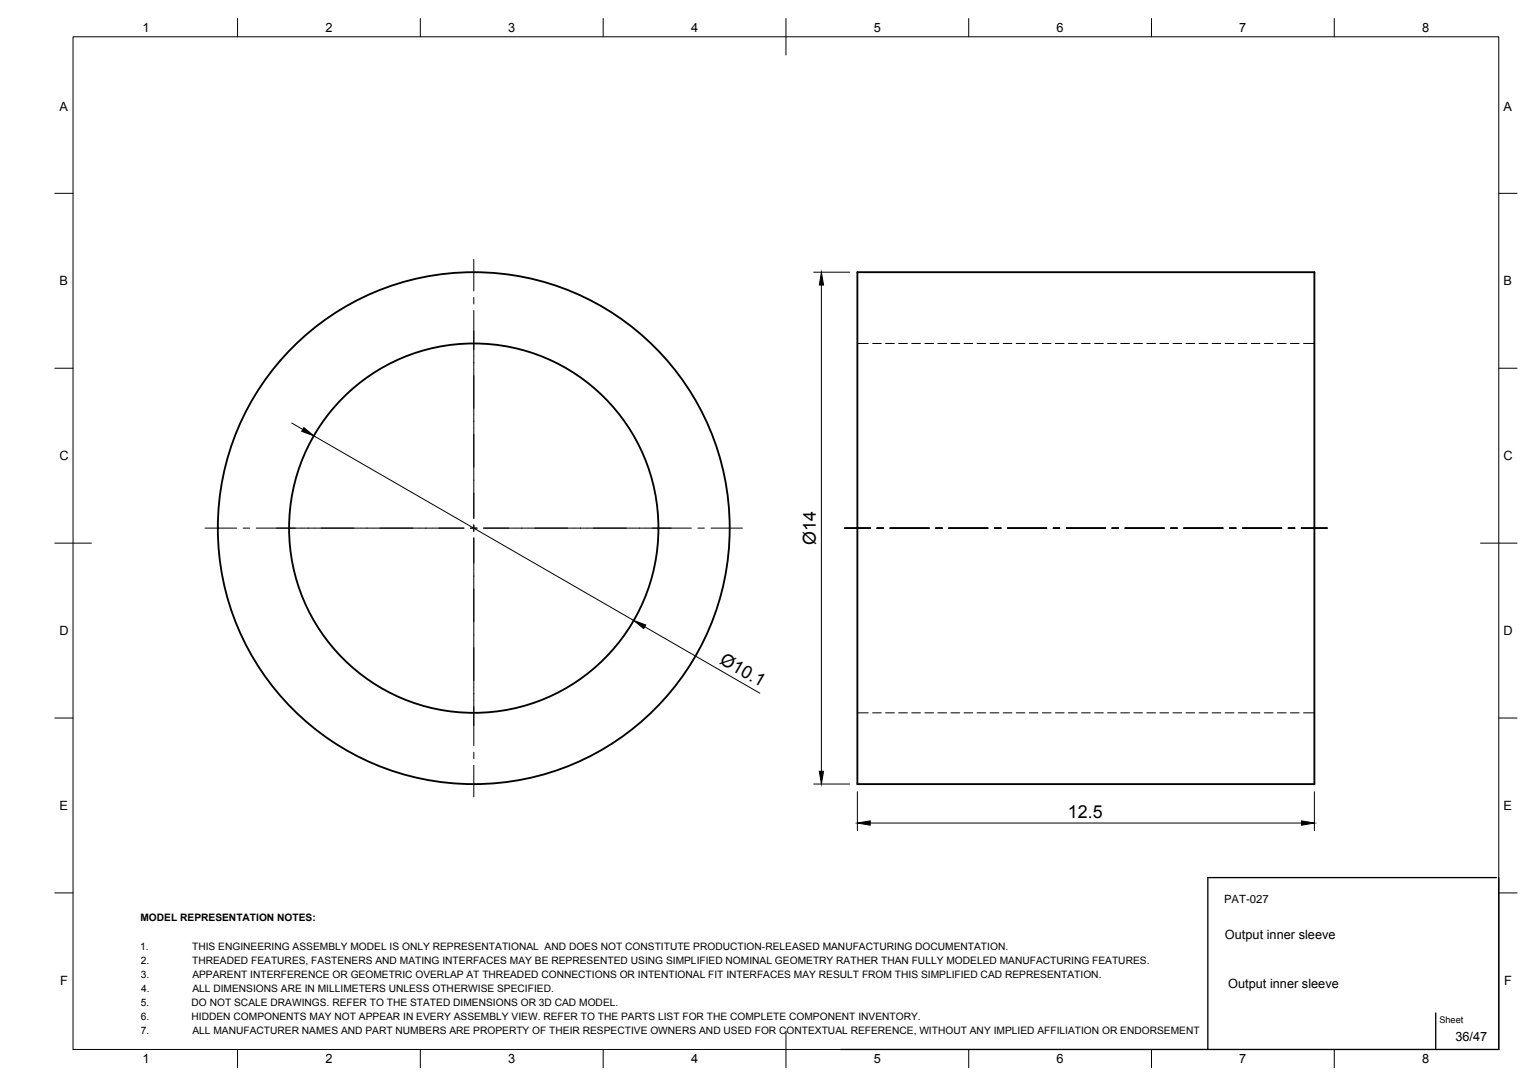
ISO-10303-21;
HEADER;
/* Generated by software containing ST-Developer
 * from STEP Tools, Inc. (www.steptools.com) 
 */

FILE_DESCRIPTION(
/* description */ ('Crank-driven oscillating fan base (mechanism only)'),

/* implementation_level */ '2;1');

FILE_NAME(
/* name */ 'Output inner sleeve.step',
/* time_stamp */ '2026-10-28T03:25:00-07:00',
/* author */ (''),
/* organization */ (''),
/* preprocessor_version */ 'ST-DEVELOPER v20.2',
/* originating_system */ 'Autodesk Translation Framework v15.17.0.0',
/* authorisation */ '');

FILE_SCHEMA (('AUTOMOTIVE_DESIGN { 1 0 10303 214 3 1 1 }'));
ENDSEC;

DATA;
#10=MECHANICAL_DESIGN_GEOMETRIC_PRESENTATION_REPRESENTATION('',(#472),#11916);
#384=SHAPE_REPRESENTATION_RELATIONSHIP('SRR','None',#12111,#424);
#424=ADVANCED_BREP_SHAPE_REPRESENTATION('',(#519),#11902);
#472=STYLED_ITEM('',(#12368),#519);
#519=MANIFOLD_SOLID_BREP('Body1',#6103);
#663=FACE_BOUND('',#1674,.T.);
#664=FACE_BOUND('',#1676,.T.);
#827=PLANE('',#7175);
#828=PLANE('',#7176);
#1163=FACE_OUTER_BOUND('',#1671,.T.);
#1164=FACE_OUTER_BOUND('',#1672,.T.);
#1165=FACE_OUTER_BOUND('',#1673,.T.);
#1166=FACE_OUTER_BOUND('',#1675,.T.);
#1671=EDGE_LOOP('',(#5194,#5195,#5196,#5197));
#1672=EDGE_LOOP('',(#5198,#5199,#5200,#5201));
#1673=EDGE_LOOP('',(#5202));
#1674=EDGE_LOOP('',(#5203));
#1675=EDGE_LOOP('',(#5204));
#1676=EDGE_LOOP('',(#5205));
#2030=LINE('',#11303,#2363);
#2031=LINE('',#11309,#2364);
#2363=VECTOR('',#8867,0.505000000000001);
#2364=VECTOR('',#8874,0.699999999999999);
#2759=CIRCLE('',#7170,0.505000000000001);
#2760=CIRCLE('',#7171,0.505000000000001);
#2761=CIRCLE('',#7173,0.699999999999999);
#2762=CIRCLE('',#7174,0.699999999999999);
#3214=VERTEX_POINT('',#11300);
#3215=VERTEX_POINT('',#11302);
#3216=VERTEX_POINT('',#11306);
#3217=VERTEX_POINT('',#11308);
#3892=EDGE_CURVE('',#3214,#3214,#2759,.T.);
#3893=EDGE_CURVE('',#3214,#3215,#2030,.T.);
#3894=EDGE_CURVE('',#3215,#3215,#2760,.T.);
#3895=EDGE_CURVE('',#3216,#3216,#2761,.T.);
#3896=EDGE_CURVE('',#3216,#3217,#2031,.T.);
#3897=EDGE_CURVE('',#3217,#3217,#2762,.T.);
#5194=ORIENTED_EDGE('',*,*,#3892,.F.);
#5195=ORIENTED_EDGE('',*,*,#3893,.T.);
#5196=ORIENTED_EDGE('',*,*,#3894,.T.);
#5197=ORIENTED_EDGE('',*,*,#3893,.F.);
#5198=ORIENTED_EDGE('',*,*,#3895,.F.);
#5199=ORIENTED_EDGE('',*,*,#3896,.T.);
#5200=ORIENTED_EDGE('',*,*,#3897,.T.);
#5201=ORIENTED_EDGE('',*,*,#3896,.F.);
#5202=ORIENTED_EDGE('',*,*,#3895,.T.);
#5203=ORIENTED_EDGE('',*,*,#3892,.T.);
#5204=ORIENTED_EDGE('',*,*,#3897,.F.);
#5205=ORIENTED_EDGE('',*,*,#3894,.F.);
#5661=CYLINDRICAL_SURFACE('',#7169,0.505000000000001);
#5662=CYLINDRICAL_SURFACE('',#7172,0.699999999999999);
#5969=ADVANCED_FACE('',(#1163),#5661,.F.);
#5970=ADVANCED_FACE('',(#1164),#5662,.T.);
#5971=ADVANCED_FACE('',(#1165,#663),#827,.T.);
#5972=ADVANCED_FACE('',(#1166,#664),#828,.F.);
#6103=CLOSED_SHELL('',(#5969,#5970,#5971,#5972));
#7168=AXIS2_PLACEMENT_3D('',#11298,#8861,#8862);
#7169=AXIS2_PLACEMENT_3D('',#11299,#8863,#8864);
#7170=AXIS2_PLACEMENT_3D('',#11301,#8865,#8866);
#7171=AXIS2_PLACEMENT_3D('',#11304,#8868,#8869);
#7172=AXIS2_PLACEMENT_3D('',#11305,#8870,#8871);
#7173=AXIS2_PLACEMENT_3D('',#11307,#8872,#8873);
#7174=AXIS2_PLACEMENT_3D('',#11310,#8875,#8876);
#7175=AXIS2_PLACEMENT_3D('',#11311,#8877,#8878);
#7176=AXIS2_PLACEMENT_3D('',#11312,#8879,#8880);
#8861=DIRECTION('axis',(0.,0.,1.));
#8862=DIRECTION('refdir',(1.,0.,0.));
#8863=DIRECTION('center_axis',(0.,0.,1.));
#8864=DIRECTION('ref_axis',(1.,0.,0.));
#8865=DIRECTION('center_axis',(0.,0.,-1.));
#8866=DIRECTION('ref_axis',(1.,0.,0.));
#8867=DIRECTION('',(0.,0.,-1.));
#8868=DIRECTION('center_axis',(0.,0.,-1.));
#8869=DIRECTION('ref_axis',(1.,0.,0.));
#8870=DIRECTION('center_axis',(0.,0.,1.));
#8871=DIRECTION('ref_axis',(1.,0.,0.));
#8872=DIRECTION('center_axis',(0.,0.,1.));
#8873=DIRECTION('ref_axis',(1.,0.,0.));
#8874=DIRECTION('',(0.,0.,-1.));
#8875=DIRECTION('center_axis',(0.,0.,1.));
#8876=DIRECTION('ref_axis',(1.,0.,0.));
#8877=DIRECTION('center_axis',(0.,0.,1.));
#8878=DIRECTION('ref_axis',(1.,0.,0.));
#8879=DIRECTION('center_axis',(0.,0.,1.));
#8880=DIRECTION('ref_axis',(1.,0.,0.));
#11298=CARTESIAN_POINT('',(0.,0.,0.));
#11299=CARTESIAN_POINT('Origin',(8.,0.,1.8));
#11300=CARTESIAN_POINT('',(7.495,-6.18446633569414E-17,3.05));
#11301=CARTESIAN_POINT('Origin',(8.,0.,3.05));
#11302=CARTESIAN_POINT('',(7.495,-6.18446633569414E-17,1.8));
#11303=CARTESIAN_POINT('',(7.495,-6.18446633569414E-17,1.8));
#11304=CARTESIAN_POINT('Origin',(8.,0.,1.8));
#11305=CARTESIAN_POINT('Origin',(8.,0.,1.8));
#11306=CARTESIAN_POINT('',(7.3,-8.57252759403146E-17,3.05));
#11307=CARTESIAN_POINT('Origin',(8.,0.,3.05));
#11308=CARTESIAN_POINT('',(7.3,-8.57252759403146E-17,1.8));
#11309=CARTESIAN_POINT('',(7.3,-8.57252759403146E-17,1.8));
#11310=CARTESIAN_POINT('Origin',(8.,0.,1.8));
#11311=CARTESIAN_POINT('Origin',(8.,0.,3.05));
#11312=CARTESIAN_POINT('Origin',(8.,0.,1.8));
#11855=UNCERTAINTY_MEASURE_WITH_UNIT(LENGTH_MEASURE(0.001),#11917,
'DISTANCE_ACCURACY_VALUE',
'Maximum model space distance between geometric entities at asserted c
onnectivities');
#11869=UNCERTAINTY_MEASURE_WITH_UNIT(LENGTH_MEASURE(0.001),#11917,
'DISTANCE_ACCURACY_VALUE',
'Maximum model space distance between geometric entities at asserted c
onnectivities');
#11902=(
GEOMETRIC_REPRESENTATION_CONTEXT(3)
GLOBAL_UNCERTAINTY_ASSIGNED_CONTEXT((#11855))
GLOBAL_UNIT_ASSIGNED_CONTEXT((#11917,#11919,#11920))
REPRESENTATION_CONTEXT('','3D')
);
#11916=(
GEOMETRIC_REPRESENTATION_CONTEXT(3)
GLOBAL_UNCERTAINTY_ASSIGNED_CONTEXT((#11869))
GLOBAL_UNIT_ASSIGNED_CONTEXT((#11917,#11919,#11920))
REPRESENTATION_CONTEXT('','3D')
);
#11917=(
LENGTH_UNIT()
NAMED_UNIT(*)
SI_UNIT(.CENTI.,.METRE.)
);
#11919=(
NAMED_UNIT(*)
PLANE_ANGLE_UNIT()
SI_UNIT($,.RADIAN.)
);
#11920=(
NAMED_UNIT(*)
SI_UNIT($,.STERADIAN.)
SOLID_ANGLE_UNIT()
);
#11953=SHAPE_DEFINITION_REPRESENTATION(#12004,#12111);
#12004=PRODUCT_DEFINITION_SHAPE('',$,#12158);
#12111=SHAPE_REPRESENTATION('',(#7168),#11902);
#12125=PRODUCT_DEFINITION_CONTEXT('part definition',#12265,'design');
#12158=PRODUCT_DEFINITION('Output inner sleeve','Output inner sleeve',#12204,
#12125);
#12204=PRODUCT_DEFINITION_FORMATION('',$,#12299);
#12265=APPLICATION_CONTEXT(
'Core Data for Automotive Mechanical Design Process');
#12266=PRODUCT_CONTEXT('part definition',#12265,'mechanical');
#12299=PRODUCT('Output inner sleeve','Output inner sleeve',
'Output inner sleeve',(#12266));
#12362=COLOUR_RGB('Sky Blue',0.24,0.69,0.87);
#12363=FILL_AREA_STYLE_COLOUR('',#12362);
#12364=FILL_AREA_STYLE('',(#12363));
#12365=SURFACE_STYLE_FILL_AREA(#12364);
#12366=SURFACE_SIDE_STYLE('',(#12365));
#12367=SURFACE_STYLE_USAGE(.BOTH.,#12366);
#12368=PRESENTATION_STYLE_ASSIGNMENT((#12367));
ENDSEC;
END-ISO-10303-21;
